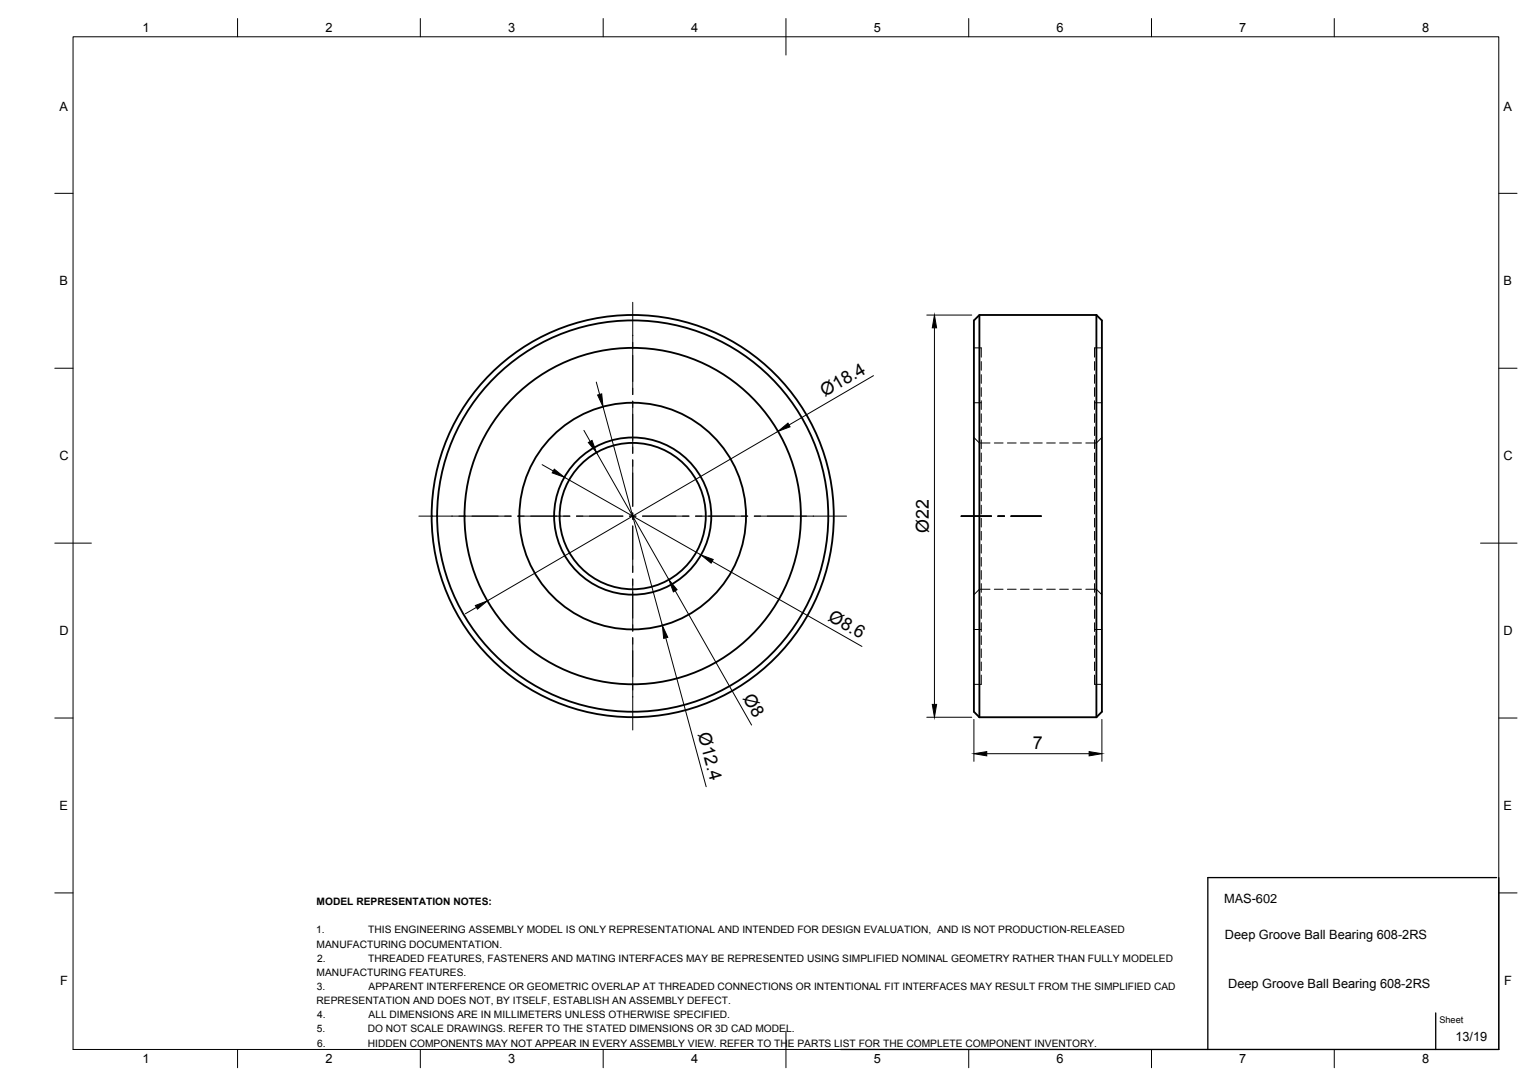
ISO-10303-21;
HEADER;
/* Generated by software containing ST-Developer
 * from STEP Tools, Inc. (www.steptools.com) 
 */

FILE_DESCRIPTION(
/* description */ (''),
/* implementation_level */ '2;1');

FILE_NAME(
/* name */ 'Deep Groove Ball Bearing 608-2RS.step',
/* time_stamp */ '2026-10-15T14:42:47-07:00',
/* author */ (''),
/* organization */ (''),
/* preprocessor_version */ 'ST-DEVELOPER v20.2',
/* originating_system */ 'Autodesk Translation Framework v15.15.0.0',
/* authorisation */ '');

FILE_SCHEMA (('AUTOMOTIVE_DESIGN { 1 0 10303 214 3 1 1 }'));
ENDSEC;

DATA;
#10=MECHANICAL_DESIGN_GEOMETRIC_PRESENTATION_REPRESENTATION('',(#241),#85789);
#165=CONICAL_SURFACE('',#10569,0.415,0.785398163397448);
#166=CONICAL_SURFACE('',#10581,1.085,0.785398163397452);
#167=CONICAL_SURFACE('',#10585,1.085,0.785398163397454);
#168=CONICAL_SURFACE('',#10597,0.415,0.785398163397449);
#205=SHAPE_REPRESENTATION_RELATIONSHIP('SRR','None',#85870,#223);
#223=ADVANCED_BREP_SHAPE_REPRESENTATION('',(#259),#85778);
#241=STYLED_ITEM('',(#85969),#259);
#259=MANIFOLD_SOLID_BREP('Body1',#9888);
#449=FACE_BOUND('',#3282,.T.);
#450=FACE_BOUND('',#3285,.T.);
#451=FACE_BOUND('',#3288,.T.);
#452=FACE_BOUND('',#3293,.T.);
#453=FACE_BOUND('',#3296,.T.);
#454=FACE_BOUND('',#3299,.T.);
#1112=PLANE('',#10571);
#1113=PLANE('',#10575);
#1114=PLANE('',#10579);
#1115=PLANE('',#10587);
#1116=PLANE('',#10591);
#1117=PLANE('',#10595);
#1529=LINE('',#77333,#2065);
#1530=LINE('',#77337,#2066);
#1531=LINE('',#77345,#2067);
#1532=LINE('',#77352,#2068);
#1533=LINE('',#77359,#2069);
#1534=LINE('',#77363,#2070);
#1535=LINE('',#77366,#2071);
#1536=LINE('',#77374,#2072);
#1537=LINE('',#77381,#2073);
#1538=LINE('',#77386,#2074);
#2065=VECTOR('',#12229,0.4);
#2066=VECTOR('',#12234,0.415);
#2067=VECTOR('',#12245,0.62);
#2068=VECTOR('',#12254,0.92);
#2069=VECTOR('',#12263,1.085);
#2070=VECTOR('',#12268,1.1);
#2071=VECTOR('',#12271,1.085);
#2072=VECTOR('',#12282,0.92);
#2073=VECTOR('',#12291,0.62);
#2074=VECTOR('',#12298,0.415);
#2338=CYLINDRICAL_SURFACE('',#10566,0.4);
#2339=CYLINDRICAL_SURFACE('',#10573,0.62);
#2340=CYLINDRICAL_SURFACE('',#10577,0.92);
#2341=CYLINDRICAL_SURFACE('',#10583,1.1);
#2342=CYLINDRICAL_SURFACE('',#10589,0.92);
#2343=CYLINDRICAL_SURFACE('',#10593,0.62);
#2715=FACE_OUTER_BOUND('',#3279,.T.);
#2716=FACE_OUTER_BOUND('',#3280,.T.);
#2717=FACE_OUTER_BOUND('',#3281,.T.);
#2718=FACE_OUTER_BOUND('',#3283,.T.);
#2719=FACE_OUTER_BOUND('',#3284,.T.);
#2720=FACE_OUTER_BOUND('',#3286,.T.);
#2721=FACE_OUTER_BOUND('',#3287,.T.);
#2722=FACE_OUTER_BOUND('',#3289,.T.);
#2723=FACE_OUTER_BOUND('',#3290,.T.);
#2724=FACE_OUTER_BOUND('',#3291,.T.);
#2725=FACE_OUTER_BOUND('',#3292,.T.);
#2726=FACE_OUTER_BOUND('',#3294,.T.);
#2727=FACE_OUTER_BOUND('',#3295,.T.);
#2728=FACE_OUTER_BOUND('',#3297,.T.);
#2729=FACE_OUTER_BOUND('',#3298,.T.);
#2730=FACE_OUTER_BOUND('',#3300,.T.);
#3279=EDGE_LOOP('',(#8411,#8412,#8413,#8414));
#3280=EDGE_LOOP('',(#8415,#8416,#8417,#8418));
#3281=EDGE_LOOP('',(#8419));
#3282=EDGE_LOOP('',(#8420));
#3283=EDGE_LOOP('',(#8421,#8422,#8423,#8424));
#3284=EDGE_LOOP('',(#8425));
#3285=EDGE_LOOP('',(#8426));
#3286=EDGE_LOOP('',(#8427,#8428,#8429,#8430));
#3287=EDGE_LOOP('',(#8431));
#3288=EDGE_LOOP('',(#8432));
#3289=EDGE_LOOP('',(#8433,#8434,#8435,#8436));
#3290=EDGE_LOOP('',(#8437,#8438,#8439,#8440));
#3291=EDGE_LOOP('',(#8441,#8442,#8443,#8444));
#3292=EDGE_LOOP('',(#8445));
#3293=EDGE_LOOP('',(#8446));
#3294=EDGE_LOOP('',(#8447,#8448,#8449,#8450));
#3295=EDGE_LOOP('',(#8451));
#3296=EDGE_LOOP('',(#8452));
#3297=EDGE_LOOP('',(#8453,#8454,#8455,#8456));
#3298=EDGE_LOOP('',(#8457));
#3299=EDGE_LOOP('',(#8458));
#3300=EDGE_LOOP('',(#8459,#8460,#8461,#8462));
#3728=CIRCLE('',#10567,0.4);
#3729=CIRCLE('',#10568,0.4);
#3730=CIRCLE('',#10570,0.43);
#3731=CIRCLE('',#10572,0.62);
#3732=CIRCLE('',#10574,0.62);
#3733=CIRCLE('',#10576,0.92);
#3734=CIRCLE('',#10578,0.92);
#3735=CIRCLE('',#10580,1.07);
#3736=CIRCLE('',#10582,1.1);
#3737=CIRCLE('',#10584,1.1);
#3738=CIRCLE('',#10586,1.07);
#3739=CIRCLE('',#10588,0.92);
#3740=CIRCLE('',#10590,0.92);
#3741=CIRCLE('',#10592,0.62);
#3742=CIRCLE('',#10594,0.62);
#3743=CIRCLE('',#10596,0.43);
#4603=VERTEX_POINT('',#77330);
#4604=VERTEX_POINT('',#77332);
#4605=VERTEX_POINT('',#77336);
#4606=VERTEX_POINT('',#77340);
#4607=VERTEX_POINT('',#77343);
#4608=VERTEX_POINT('',#77347);
#4609=VERTEX_POINT('',#77350);
#4610=VERTEX_POINT('',#77354);
#4611=VERTEX_POINT('',#77357);
#4612=VERTEX_POINT('',#77361);
#4613=VERTEX_POINT('',#77365);
#4614=VERTEX_POINT('',#77369);
#4615=VERTEX_POINT('',#77372);
#4616=VERTEX_POINT('',#77376);
#4617=VERTEX_POINT('',#77379);
#4618=VERTEX_POINT('',#77383);
#5933=EDGE_CURVE('',#4603,#4603,#3728,.T.);
#5934=EDGE_CURVE('',#4603,#4604,#1529,.T.);
#5935=EDGE_CURVE('',#4604,#4604,#3729,.T.);
#5936=EDGE_CURVE('',#4603,#4605,#1530,.T.);
#5937=EDGE_CURVE('',#4605,#4605,#3730,.T.);
#5938=EDGE_CURVE('',#4606,#4606,#3731,.T.);
#5939=EDGE_CURVE('',#4607,#4607,#3732,.T.);
#5940=EDGE_CURVE('',#4607,#4606,#1531,.T.);
#5941=EDGE_CURVE('',#4608,#4608,#3733,.T.);
#5942=EDGE_CURVE('',#4609,#4609,#3734,.T.);
#5943=EDGE_CURVE('',#4609,#4608,#1532,.T.);
#5944=EDGE_CURVE('',#4610,#4610,#3735,.T.);
#5945=EDGE_CURVE('',#4611,#4611,#3736,.T.);
#5946=EDGE_CURVE('',#4611,#4610,#1533,.T.);
#5947=EDGE_CURVE('',#4612,#4612,#3737,.T.);
#5948=EDGE_CURVE('',#4612,#4611,#1534,.T.);
#5949=EDGE_CURVE('',#4612,#4613,#1535,.T.);
#5950=EDGE_CURVE('',#4613,#4613,#3738,.T.);
#5951=EDGE_CURVE('',#4614,#4614,#3739,.T.);
#5952=EDGE_CURVE('',#4615,#4615,#3740,.T.);
#5953=EDGE_CURVE('',#4615,#4614,#1536,.T.);
#5954=EDGE_CURVE('',#4616,#4616,#3741,.T.);
#5955=EDGE_CURVE('',#4617,#4617,#3742,.T.);
#5956=EDGE_CURVE('',#4617,#4616,#1537,.T.);
#5957=EDGE_CURVE('',#4618,#4618,#3743,.T.);
#5958=EDGE_CURVE('',#4604,#4618,#1538,.T.);
#8411=ORIENTED_EDGE('',*,*,#5933,.F.);
#8412=ORIENTED_EDGE('',*,*,#5934,.T.);
#8413=ORIENTED_EDGE('',*,*,#5935,.T.);
#8414=ORIENTED_EDGE('',*,*,#5934,.F.);
#8415=ORIENTED_EDGE('',*,*,#5933,.T.);
#8416=ORIENTED_EDGE('',*,*,#5936,.T.);
#8417=ORIENTED_EDGE('',*,*,#5937,.F.);
#8418=ORIENTED_EDGE('',*,*,#5936,.F.);
#8419=ORIENTED_EDGE('',*,*,#5938,.F.);
#8420=ORIENTED_EDGE('',*,*,#5937,.T.);
#8421=ORIENTED_EDGE('',*,*,#5939,.F.);
#8422=ORIENTED_EDGE('',*,*,#5940,.T.);
#8423=ORIENTED_EDGE('',*,*,#5938,.T.);
#8424=ORIENTED_EDGE('',*,*,#5940,.F.);
#8425=ORIENTED_EDGE('',*,*,#5941,.F.);
#8426=ORIENTED_EDGE('',*,*,#5939,.T.);
#8427=ORIENTED_EDGE('',*,*,#5942,.F.);
#8428=ORIENTED_EDGE('',*,*,#5943,.T.);
#8429=ORIENTED_EDGE('',*,*,#5941,.T.);
#8430=ORIENTED_EDGE('',*,*,#5943,.F.);
#8431=ORIENTED_EDGE('',*,*,#5944,.F.);
#8432=ORIENTED_EDGE('',*,*,#5942,.T.);
#8433=ORIENTED_EDGE('',*,*,#5945,.F.);
#8434=ORIENTED_EDGE('',*,*,#5946,.T.);
#8435=ORIENTED_EDGE('',*,*,#5944,.T.);
#8436=ORIENTED_EDGE('',*,*,#5946,.F.);
#8437=ORIENTED_EDGE('',*,*,#5947,.F.);
#8438=ORIENTED_EDGE('',*,*,#5948,.T.);
#8439=ORIENTED_EDGE('',*,*,#5945,.T.);
#8440=ORIENTED_EDGE('',*,*,#5948,.F.);
#8441=ORIENTED_EDGE('',*,*,#5947,.T.);
#8442=ORIENTED_EDGE('',*,*,#5949,.T.);
#8443=ORIENTED_EDGE('',*,*,#5950,.F.);
#8444=ORIENTED_EDGE('',*,*,#5949,.F.);
#8445=ORIENTED_EDGE('',*,*,#5950,.T.);
#8446=ORIENTED_EDGE('',*,*,#5951,.F.);
#8447=ORIENTED_EDGE('',*,*,#5952,.F.);
#8448=ORIENTED_EDGE('',*,*,#5953,.T.);
#8449=ORIENTED_EDGE('',*,*,#5951,.T.);
#8450=ORIENTED_EDGE('',*,*,#5953,.F.);
#8451=ORIENTED_EDGE('',*,*,#5952,.T.);
#8452=ORIENTED_EDGE('',*,*,#5954,.F.);
#8453=ORIENTED_EDGE('',*,*,#5955,.F.);
#8454=ORIENTED_EDGE('',*,*,#5956,.T.);
#8455=ORIENTED_EDGE('',*,*,#5954,.T.);
#8456=ORIENTED_EDGE('',*,*,#5956,.F.);
#8457=ORIENTED_EDGE('',*,*,#5955,.T.);
#8458=ORIENTED_EDGE('',*,*,#5957,.F.);
#8459=ORIENTED_EDGE('',*,*,#5935,.F.);
#8460=ORIENTED_EDGE('',*,*,#5958,.T.);
#8461=ORIENTED_EDGE('',*,*,#5957,.T.);
#8462=ORIENTED_EDGE('',*,*,#5958,.F.);
#9693=ADVANCED_FACE('',(#2715),#2338,.F.);
#9694=ADVANCED_FACE('',(#2716),#165,.F.);
#9695=ADVANCED_FACE('',(#2717,#449),#1112,.T.);
#9696=ADVANCED_FACE('',(#2718),#2339,.T.);
#9697=ADVANCED_FACE('',(#2719,#450),#1113,.T.);
#9698=ADVANCED_FACE('',(#2720),#2340,.F.);
#9699=ADVANCED_FACE('',(#2721,#451),#1114,.T.);
#9700=ADVANCED_FACE('',(#2722),#166,.T.);
#9701=ADVANCED_FACE('',(#2723),#2341,.T.);
#9702=ADVANCED_FACE('',(#2724),#167,.T.);
#9703=ADVANCED_FACE('',(#2725,#452),#1115,.T.);
#9704=ADVANCED_FACE('',(#2726),#2342,.F.);
#9705=ADVANCED_FACE('',(#2727,#453),#1116,.T.);
#9706=ADVANCED_FACE('',(#2728),#2343,.T.);
#9707=ADVANCED_FACE('',(#2729,#454),#1117,.T.);
#9708=ADVANCED_FACE('',(#2730),#168,.F.);
#9888=CLOSED_SHELL('',(#9693,#9694,#9695,#9696,#9697,#9698,#9699,#9700,
#9701,#9702,#9703,#9704,#9705,#9706,#9707,#9708));
#10565=AXIS2_PLACEMENT_3D('',#77328,#12223,#12224);
#10566=AXIS2_PLACEMENT_3D('',#77329,#12225,#12226);
#10567=AXIS2_PLACEMENT_3D('',#77331,#12227,#12228);
#10568=AXIS2_PLACEMENT_3D('',#77334,#12230,#12231);
#10569=AXIS2_PLACEMENT_3D('',#77335,#12232,#12233);
#10570=AXIS2_PLACEMENT_3D('',#77338,#12235,#12236);
#10571=AXIS2_PLACEMENT_3D('',#77339,#12237,#12238);
#10572=AXIS2_PLACEMENT_3D('',#77341,#12239,#12240);
#10573=AXIS2_PLACEMENT_3D('',#77342,#12241,#12242);
#10574=AXIS2_PLACEMENT_3D('',#77344,#12243,#12244);
#10575=AXIS2_PLACEMENT_3D('',#77346,#12246,#12247);
#10576=AXIS2_PLACEMENT_3D('',#77348,#12248,#12249);
#10577=AXIS2_PLACEMENT_3D('',#77349,#12250,#12251);
#10578=AXIS2_PLACEMENT_3D('',#77351,#12252,#12253);
#10579=AXIS2_PLACEMENT_3D('',#77353,#12255,#12256);
#10580=AXIS2_PLACEMENT_3D('',#77355,#12257,#12258);
#10581=AXIS2_PLACEMENT_3D('',#77356,#12259,#12260);
#10582=AXIS2_PLACEMENT_3D('',#77358,#12261,#12262);
#10583=AXIS2_PLACEMENT_3D('',#77360,#12264,#12265);
#10584=AXIS2_PLACEMENT_3D('',#77362,#12266,#12267);
#10585=AXIS2_PLACEMENT_3D('',#77364,#12269,#12270);
#10586=AXIS2_PLACEMENT_3D('',#77367,#12272,#12273);
#10587=AXIS2_PLACEMENT_3D('',#77368,#12274,#12275);
#10588=AXIS2_PLACEMENT_3D('',#77370,#12276,#12277);
#10589=AXIS2_PLACEMENT_3D('',#77371,#12278,#12279);
#10590=AXIS2_PLACEMENT_3D('',#77373,#12280,#12281);
#10591=AXIS2_PLACEMENT_3D('',#77375,#12283,#12284);
#10592=AXIS2_PLACEMENT_3D('',#77377,#12285,#12286);
#10593=AXIS2_PLACEMENT_3D('',#77378,#12287,#12288);
#10594=AXIS2_PLACEMENT_3D('',#77380,#12289,#12290);
#10595=AXIS2_PLACEMENT_3D('',#77382,#12292,#12293);
#10596=AXIS2_PLACEMENT_3D('',#77384,#12294,#12295);
#10597=AXIS2_PLACEMENT_3D('',#77385,#12296,#12297);
#12223=DIRECTION('axis',(0.,0.,1.));
#12224=DIRECTION('refdir',(1.,0.,0.));
#12225=DIRECTION('center_axis',(0.,0.,1.));
#12226=DIRECTION('ref_axis',(1.,0.,0.));
#12227=DIRECTION('center_axis',(0.,0.,1.));
#12228=DIRECTION('ref_axis',(1.,0.,0.));
#12229=DIRECTION('',(0.,0.,1.));
#12230=DIRECTION('center_axis',(0.,0.,1.));
#12231=DIRECTION('ref_axis',(1.,0.,0.));
#12232=DIRECTION('center_axis',(0.,0.,-1.));
#12233=DIRECTION('ref_axis',(1.,0.,0.));
#12234=DIRECTION('',(-0.707106781186547,8.65956056235493E-17,-0.707106781186548));
#12235=DIRECTION('center_axis',(0.,0.,1.));
#12236=DIRECTION('ref_axis',(1.,0.,0.));
#12237=DIRECTION('center_axis',(0.,0.,-1.));
#12238=DIRECTION('ref_axis',(-1.,0.,0.));
#12239=DIRECTION('center_axis',(0.,0.,1.));
#12240=DIRECTION('ref_axis',(1.,0.,0.));
#12241=DIRECTION('center_axis',(0.,0.,1.));
#12242=DIRECTION('ref_axis',(1.,0.,0.));
#12243=DIRECTION('center_axis',(0.,0.,1.));
#12244=DIRECTION('ref_axis',(1.,0.,0.));
#12245=DIRECTION('',(0.,0.,-1.));
#12246=DIRECTION('center_axis',(0.,0.,-1.));
#12247=DIRECTION('ref_axis',(-1.,0.,0.));
#12248=DIRECTION('center_axis',(0.,0.,1.));
#12249=DIRECTION('ref_axis',(1.,0.,0.));
#12250=DIRECTION('center_axis',(0.,0.,1.));
#12251=DIRECTION('ref_axis',(1.,0.,0.));
#12252=DIRECTION('center_axis',(0.,0.,1.));
#12253=DIRECTION('ref_axis',(1.,0.,0.));
#12254=DIRECTION('',(0.,0.,1.));
#12255=DIRECTION('center_axis',(0.,0.,-1.));
#12256=DIRECTION('ref_axis',(-1.,0.,0.));
#12257=DIRECTION('center_axis',(0.,0.,1.));
#12258=DIRECTION('ref_axis',(1.,0.,0.));
#12259=DIRECTION('center_axis',(0.,0.,1.));
#12260=DIRECTION('ref_axis',(1.,0.,0.));
#12261=DIRECTION('center_axis',(0.,0.,1.));
#12262=DIRECTION('ref_axis',(1.,0.,0.));
#12263=DIRECTION('',(0.70710678118655,8.65956056235497E-17,-0.707106781186545));
#12264=DIRECTION('center_axis',(0.,0.,1.));
#12265=DIRECTION('ref_axis',(1.,0.,0.));
#12266=DIRECTION('center_axis',(0.,0.,1.));
#12267=DIRECTION('ref_axis',(1.,0.,0.));
#12268=DIRECTION('',(0.,0.,-1.));
#12269=DIRECTION('center_axis',(0.,0.,-1.));
#12270=DIRECTION('ref_axis',(1.,0.,0.));
#12271=DIRECTION('',(0.707106781186552,-8.65956056235498E-17,0.707106781186543));
#12272=DIRECTION('center_axis',(0.,0.,1.));
#12273=DIRECTION('ref_axis',(1.,0.,0.));
#12274=DIRECTION('center_axis',(0.,0.,1.));
#12275=DIRECTION('ref_axis',(1.,0.,0.));
#12276=DIRECTION('center_axis',(0.,0.,1.));
#12277=DIRECTION('ref_axis',(1.,0.,0.));
#12278=DIRECTION('center_axis',(0.,0.,1.));
#12279=DIRECTION('ref_axis',(1.,0.,0.));
#12280=DIRECTION('center_axis',(0.,0.,1.));
#12281=DIRECTION('ref_axis',(1.,0.,0.));
#12282=DIRECTION('',(0.,0.,1.));
#12283=DIRECTION('center_axis',(0.,0.,1.));
#12284=DIRECTION('ref_axis',(1.,0.,0.));
#12285=DIRECTION('center_axis',(0.,0.,1.));
#12286=DIRECTION('ref_axis',(1.,0.,0.));
#12287=DIRECTION('center_axis',(0.,0.,1.));
#12288=DIRECTION('ref_axis',(1.,0.,0.));
#12289=DIRECTION('center_axis',(0.,0.,1.));
#12290=DIRECTION('ref_axis',(1.,0.,0.));
#12291=DIRECTION('',(0.,0.,-1.));
#12292=DIRECTION('center_axis',(0.,0.,1.));
#12293=DIRECTION('ref_axis',(1.,0.,0.));
#12294=DIRECTION('center_axis',(0.,0.,1.));
#12295=DIRECTION('ref_axis',(1.,0.,0.));
#12296=DIRECTION('center_axis',(0.,0.,1.));
#12297=DIRECTION('ref_axis',(1.,0.,0.));
#12298=DIRECTION('',(-0.707106781186548,-8.65956056235494E-17,0.707106781186547));
#77328=CARTESIAN_POINT('',(0.,0.,0.));
#77329=CARTESIAN_POINT('Origin',(0.,0.,0.35));
#77330=CARTESIAN_POINT('',(-0.4,-4.89858719658941E-17,0.03));
#77331=CARTESIAN_POINT('Origin',(0.,0.,0.03));
#77332=CARTESIAN_POINT('',(-0.4,-4.89858719658941E-17,0.67));
#77333=CARTESIAN_POINT('',(-0.4,-4.89858719658941E-17,0.35));
#77334=CARTESIAN_POINT('Origin',(0.,0.,0.67));
#77335=CARTESIAN_POINT('Origin',(0.,0.,0.015));
#77336=CARTESIAN_POINT('',(-0.43,-5.26598123633362E-17,8.67361737988404E-18));
#77337=CARTESIAN_POINT('',(-0.415,5.08228421646152E-17,0.015));
#77338=CARTESIAN_POINT('Origin',(0.,0.,0.));
#77339=CARTESIAN_POINT('Origin',(0.62,0.,0.));
#77340=CARTESIAN_POINT('',(-0.62,-7.59281015471359E-17,0.));
#77341=CARTESIAN_POINT('Origin',(0.,0.,0.));
#77342=CARTESIAN_POINT('Origin',(0.,0.,0.02));
#77343=CARTESIAN_POINT('',(-0.62,-7.59281015471359E-17,0.04));
#77344=CARTESIAN_POINT('Origin',(0.,0.,0.04));
#77345=CARTESIAN_POINT('',(-0.62,-7.59281015471359E-17,0.02));
#77346=CARTESIAN_POINT('Origin',(0.92,0.,0.04));
#77347=CARTESIAN_POINT('',(-0.92,-1.12667505521556E-16,0.04));
#77348=CARTESIAN_POINT('Origin',(0.,0.,0.04));
#77349=CARTESIAN_POINT('Origin',(0.,0.,0.02));
#77350=CARTESIAN_POINT('',(-0.92,-1.12667505521556E-16,0.));
#77351=CARTESIAN_POINT('Origin',(0.,0.,0.));
#77352=CARTESIAN_POINT('',(-0.92,-1.12667505521556E-16,0.02));
#77353=CARTESIAN_POINT('Origin',(1.07,0.,0.));
#77354=CARTESIAN_POINT('',(-1.07,-1.31037207508767E-16,6.93889390390723E-18));
#77355=CARTESIAN_POINT('Origin',(0.,0.,0.));
#77356=CARTESIAN_POINT('Origin',(0.,0.,0.015));
#77357=CARTESIAN_POINT('',(-1.1,-1.34711147906209E-16,0.03));
#77358=CARTESIAN_POINT('Origin',(0.,0.,0.03));
#77359=CARTESIAN_POINT('',(-1.085,-1.32874177707488E-16,0.015));
#77360=CARTESIAN_POINT('Origin',(0.,0.,0.35));
#77361=CARTESIAN_POINT('',(-1.1,-1.34711147906209E-16,0.67));
#77362=CARTESIAN_POINT('Origin',(0.,0.,0.67));
#77363=CARTESIAN_POINT('',(-1.1,-1.34711147906209E-16,0.35));
#77364=CARTESIAN_POINT('Origin',(0.,0.,0.685));
#77365=CARTESIAN_POINT('',(-1.07,-1.31037207508767E-16,0.7));
#77366=CARTESIAN_POINT('',(-1.085,1.32874177707488E-16,0.685));
#77367=CARTESIAN_POINT('Origin',(0.,0.,0.7));
#77368=CARTESIAN_POINT('Origin',(0.92,0.,0.7));
#77369=CARTESIAN_POINT('',(-0.92,-1.12667505521556E-16,0.7));
#77370=CARTESIAN_POINT('Origin',(0.,0.,0.7));
#77371=CARTESIAN_POINT('Origin',(0.,0.,0.68));
#77372=CARTESIAN_POINT('',(-0.92,-1.12667505521556E-16,0.66));
#77373=CARTESIAN_POINT('Origin',(0.,0.,0.66));
#77374=CARTESIAN_POINT('',(-0.92,-1.12667505521556E-16,0.68));
#77375=CARTESIAN_POINT('Origin',(0.62,0.,0.66));
#77376=CARTESIAN_POINT('',(-0.62,-7.59281015471359E-17,0.66));
#77377=CARTESIAN_POINT('Origin',(0.,0.,0.66));
#77378=CARTESIAN_POINT('Origin',(0.,0.,0.68));
#77379=CARTESIAN_POINT('',(-0.62,-7.59281015471359E-17,0.7));
#77380=CARTESIAN_POINT('Origin',(0.,0.,0.7));
#77381=CARTESIAN_POINT('',(-0.62,-7.59281015471359E-17,0.68));
#77382=CARTESIAN_POINT('Origin',(0.43,0.,0.7));
#77383=CARTESIAN_POINT('',(-0.43,-5.26598123633362E-17,0.7));
#77384=CARTESIAN_POINT('Origin',(0.,0.,0.7));
#77385=CARTESIAN_POINT('Origin',(0.,0.,0.685));
#77386=CARTESIAN_POINT('',(-0.415,-5.08228421646152E-17,0.685));
#85758=UNCERTAINTY_MEASURE_WITH_UNIT(LENGTH_MEASURE(0.001),#85790,
'DISTANCE_ACCURACY_VALUE',
'Maximum model space distance between geometric entities at asserted c
onnectivities');
#85769=UNCERTAINTY_MEASURE_WITH_UNIT(LENGTH_MEASURE(0.001),#85790,
'DISTANCE_ACCURACY_VALUE',
'Maximum model space distance between geometric entities at asserted c
onnectivities');
#85778=(
GEOMETRIC_REPRESENTATION_CONTEXT(3)
GLOBAL_UNCERTAINTY_ASSIGNED_CONTEXT((#85758))
GLOBAL_UNIT_ASSIGNED_CONTEXT((#85790,#85792,#85793))
REPRESENTATION_CONTEXT('','3D')
);
#85789=(
GEOMETRIC_REPRESENTATION_CONTEXT(3)
GLOBAL_UNCERTAINTY_ASSIGNED_CONTEXT((#85769))
GLOBAL_UNIT_ASSIGNED_CONTEXT((#85790,#85792,#85793))
REPRESENTATION_CONTEXT('','3D')
);
#85790=(
LENGTH_UNIT()
NAMED_UNIT(*)
SI_UNIT(.CENTI.,.METRE.)
);
#85792=(
NAMED_UNIT(*)
PLANE_ANGLE_UNIT()
SI_UNIT($,.RADIAN.)
);
#85793=(
NAMED_UNIT(*)
SI_UNIT($,.STERADIAN.)
SOLID_ANGLE_UNIT()
);
#85802=SHAPE_DEFINITION_REPRESENTATION(#85821,#85870);
#85821=PRODUCT_DEFINITION_SHAPE('',$,#85890);
#85870=SHAPE_REPRESENTATION('',(#10565),#85778);
#85881=PRODUCT_DEFINITION_CONTEXT('part definition',#85940,'design');
#85890=PRODUCT_DEFINITION('Deep Groove Ball Bearing 608-2RS',
'Deep Groove Ball Bearing 608-2RS',#85909,#85881);
#85909=PRODUCT_DEFINITION_FORMATION('',$,#85950);
#85940=APPLICATION_CONTEXT(
'Core Data for Automotive Mechanical Design Process');
#85941=PRODUCT_CONTEXT('part definition',#85940,'mechanical');
#85950=PRODUCT('Deep Groove Ball Bearing 608-2RS',
'Deep Groove Ball Bearing 608-2RS',$,(#85941));
#85969=PRESENTATION_STYLE_ASSIGNMENT((#85987));
#85987=SURFACE_STYLE_USAGE(.BOTH.,#86005);
#86005=SURFACE_SIDE_STYLE('',(#86023));
#86023=SURFACE_STYLE_FILL_AREA(#86041);
#86041=FILL_AREA_STYLE('Opaque(218,221,226)',(#86059));
#86059=FILL_AREA_STYLE_COLOUR('Opaque(218,221,226)',#86077);
#86077=COLOUR_RGB('Opaque(218,221,226)', 0.31764706, 0.68627451, 0.89019608);
ENDSEC;
END-ISO-10303-21;
